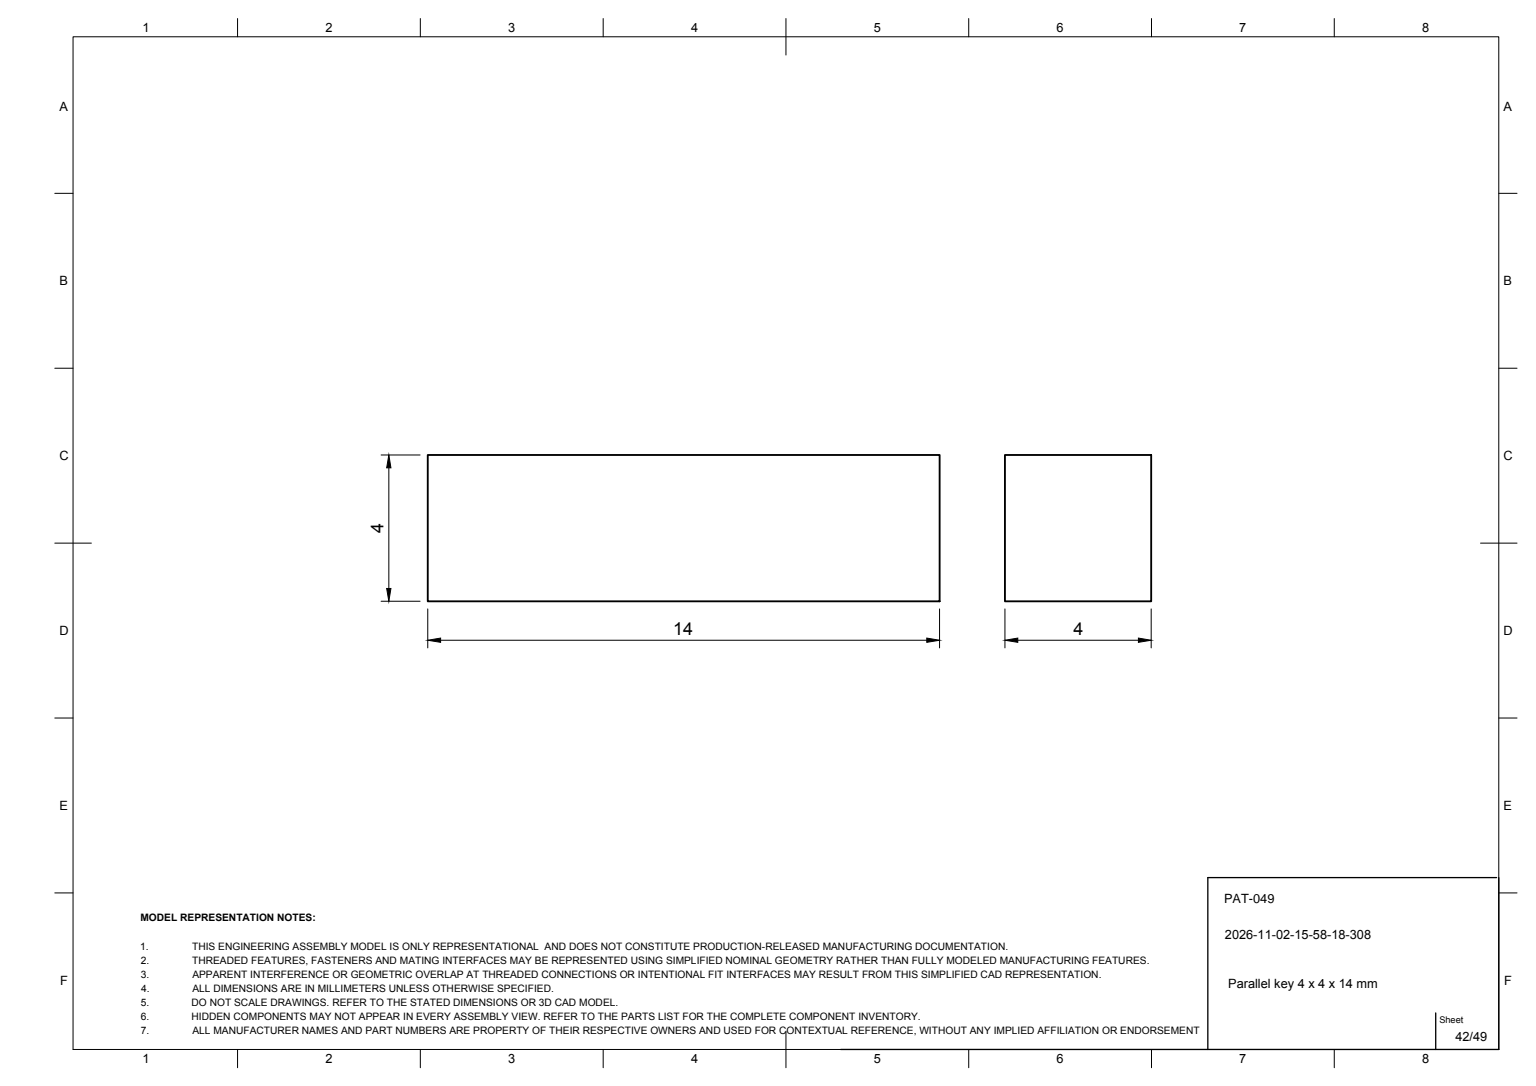
ISO-10303-21;
HEADER;
/* Generated by software containing ST-Developer
 * from STEP Tools, Inc. (www.steptools.com) 
 */

FILE_DESCRIPTION(
/* description */ ('Hand drill press frame (manual)'),
/* implementation_level */ '2;1');

FILE_NAME(
/* name */ 'Parallel key 4 x 4 x 14 mm.step',
/* time_stamp */ '2026-10-28T03:25:28-07:00',
/* author */ (''),
/* organization */ (''),
/* preprocessor_version */ 'ST-DEVELOPER v20.2',
/* originating_system */ 'Autodesk Translation Framework v15.17.0.0',
/* authorisation */ '');

FILE_SCHEMA (('AUTOMOTIVE_DESIGN { 1 0 10303 214 3 1 1 }'));
ENDSEC;

DATA;
#10=MECHANICAL_DESIGN_GEOMETRIC_PRESENTATION_REPRESENTATION('',(#660),#33299);
#563=SHAPE_REPRESENTATION_RELATIONSHIP('SRR','None',#33525,#608);
#608=ADVANCED_BREP_SHAPE_REPRESENTATION('',(#711),#33287);
#660=STYLED_ITEM('',(#33814),#711);
#711=MANIFOLD_SOLID_BREP('Body1',#12679);
#1260=PLANE('',#14070);
#1261=PLANE('',#14071);
#1262=PLANE('',#14072);
#1263=PLANE('',#14073);
#1264=PLANE('',#14074);
#1265=PLANE('',#14075);
#1861=FACE_OUTER_BOUND('',#2697,.T.);
#1862=FACE_OUTER_BOUND('',#2698,.T.);
#1863=FACE_OUTER_BOUND('',#2699,.T.);
#1864=FACE_OUTER_BOUND('',#2700,.T.);
#1865=FACE_OUTER_BOUND('',#2701,.T.);
#1866=FACE_OUTER_BOUND('',#2702,.T.);
#2697=EDGE_LOOP('',(#10979,#10980,#10981,#10982));
#2698=EDGE_LOOP('',(#10983,#10984,#10985,#10986));
#2699=EDGE_LOOP('',(#10987,#10988,#10989,#10990));
#2700=EDGE_LOOP('',(#10991,#10992,#10993,#10994));
#2701=EDGE_LOOP('',(#10995,#10996,#10997,#10998));
#2702=EDGE_LOOP('',(#10999,#11000,#11001,#11002));
#3816=LINE('',#21203,#4981);
#3817=LINE('',#21205,#4982);
#3818=LINE('',#21207,#4983);
#3819=LINE('',#21208,#4984);
#3820=LINE('',#21211,#4985);
#3821=LINE('',#21213,#4986);
#3822=LINE('',#21214,#4987);
#3823=LINE('',#21217,#4988);
#3824=LINE('',#21219,#4989);
#3825=LINE('',#21220,#4990);
#3826=LINE('',#21222,#4991);
#3827=LINE('',#21223,#4992);
#4981=VECTOR('',#17065,1.);
#4982=VECTOR('',#17066,1.);
#4983=VECTOR('',#17067,1.);
#4984=VECTOR('',#17068,1.);
#4985=VECTOR('',#17071,1.);
#4986=VECTOR('',#17072,1.);
#4987=VECTOR('',#17073,1.);
#4988=VECTOR('',#17076,1.);
#4989=VECTOR('',#17077,1.);
#4990=VECTOR('',#17078,1.);
#4991=VECTOR('',#17081,1.);
#4992=VECTOR('',#17082,1.);
#6473=VERTEX_POINT('',#21201);
#6474=VERTEX_POINT('',#21202);
#6475=VERTEX_POINT('',#21204);
#6476=VERTEX_POINT('',#21206);
#6477=VERTEX_POINT('',#21210);
#6478=VERTEX_POINT('',#21212);
#6479=VERTEX_POINT('',#21216);
#6480=VERTEX_POINT('',#21218);
#8018=EDGE_CURVE('',#6473,#6474,#3816,.T.);
#8019=EDGE_CURVE('',#6474,#6475,#3817,.T.);
#8020=EDGE_CURVE('',#6476,#6475,#3818,.T.);
#8021=EDGE_CURVE('',#6473,#6476,#3819,.T.);
#8022=EDGE_CURVE('',#6477,#6473,#3820,.T.);
#8023=EDGE_CURVE('',#6478,#6476,#3821,.T.);
#8024=EDGE_CURVE('',#6477,#6478,#3822,.T.);
#8025=EDGE_CURVE('',#6479,#6477,#3823,.T.);
#8026=EDGE_CURVE('',#6480,#6478,#3824,.T.);
#8027=EDGE_CURVE('',#6479,#6480,#3825,.T.);
#8028=EDGE_CURVE('',#6474,#6479,#3826,.T.);
#8029=EDGE_CURVE('',#6475,#6480,#3827,.T.);
#10979=ORIENTED_EDGE('',*,*,#8018,.T.);
#10980=ORIENTED_EDGE('',*,*,#8019,.T.);
#10981=ORIENTED_EDGE('',*,*,#8020,.F.);
#10982=ORIENTED_EDGE('',*,*,#8021,.F.);
#10983=ORIENTED_EDGE('',*,*,#8022,.T.);
#10984=ORIENTED_EDGE('',*,*,#8021,.T.);
#10985=ORIENTED_EDGE('',*,*,#8023,.F.);
#10986=ORIENTED_EDGE('',*,*,#8024,.F.);
#10987=ORIENTED_EDGE('',*,*,#8025,.T.);
#10988=ORIENTED_EDGE('',*,*,#8024,.T.);
#10989=ORIENTED_EDGE('',*,*,#8026,.F.);
#10990=ORIENTED_EDGE('',*,*,#8027,.F.);
#10991=ORIENTED_EDGE('',*,*,#8028,.T.);
#10992=ORIENTED_EDGE('',*,*,#8027,.T.);
#10993=ORIENTED_EDGE('',*,*,#8029,.F.);
#10994=ORIENTED_EDGE('',*,*,#8019,.F.);
#10995=ORIENTED_EDGE('',*,*,#8029,.T.);
#10996=ORIENTED_EDGE('',*,*,#8026,.T.);
#10997=ORIENTED_EDGE('',*,*,#8023,.T.);
#10998=ORIENTED_EDGE('',*,*,#8020,.T.);
#10999=ORIENTED_EDGE('',*,*,#8028,.F.);
#11000=ORIENTED_EDGE('',*,*,#8018,.F.);
#11001=ORIENTED_EDGE('',*,*,#8022,.F.);
#11002=ORIENTED_EDGE('',*,*,#8025,.F.);
#12470=ADVANCED_FACE('',(#1861),#1260,.T.);
#12471=ADVANCED_FACE('',(#1862),#1261,.T.);
#12472=ADVANCED_FACE('',(#1863),#1262,.T.);
#12473=ADVANCED_FACE('',(#1864),#1263,.T.);
#12474=ADVANCED_FACE('',(#1865),#1264,.T.);
#12475=ADVANCED_FACE('',(#1866),#1265,.F.);
#12679=CLOSED_SHELL('',(#12470,#12471,#12472,#12473,#12474,#12475));
#14069=AXIS2_PLACEMENT_3D('',#21199,#17061,#17062);
#14070=AXIS2_PLACEMENT_3D('',#21200,#17063,#17064);
#14071=AXIS2_PLACEMENT_3D('',#21209,#17069,#17070);
#14072=AXIS2_PLACEMENT_3D('',#21215,#17074,#17075);
#14073=AXIS2_PLACEMENT_3D('',#21221,#17079,#17080);
#14074=AXIS2_PLACEMENT_3D('',#21224,#17083,#17084);
#14075=AXIS2_PLACEMENT_3D('',#21225,#17085,#17086);
#17061=DIRECTION('axis',(0.,0.,1.));
#17062=DIRECTION('refdir',(1.,0.,0.));
#17063=DIRECTION('center_axis',(0.,1.,0.));
#17064=DIRECTION('ref_axis',(-1.,0.,0.));
#17065=DIRECTION('',(-1.,0.,0.));
#17066=DIRECTION('',(0.,0.,1.));
#17067=DIRECTION('',(-1.,0.,0.));
#17068=DIRECTION('',(0.,0.,1.));
#17069=DIRECTION('center_axis',(1.,0.,0.));
#17070=DIRECTION('ref_axis',(0.,1.,0.));
#17071=DIRECTION('',(0.,1.,0.));
#17072=DIRECTION('',(0.,1.,0.));
#17073=DIRECTION('',(0.,0.,1.));
#17074=DIRECTION('center_axis',(0.,-1.,0.));
#17075=DIRECTION('ref_axis',(1.,0.,0.));
#17076=DIRECTION('',(1.,0.,0.));
#17077=DIRECTION('',(1.,0.,0.));
#17078=DIRECTION('',(0.,0.,1.));
#17079=DIRECTION('center_axis',(-1.,0.,0.));
#17080=DIRECTION('ref_axis',(0.,-1.,0.));
#17081=DIRECTION('',(0.,-1.,0.));
#17082=DIRECTION('',(0.,-1.,0.));
#17083=DIRECTION('center_axis',(0.,0.,1.));
#17084=DIRECTION('ref_axis',(1.,0.,0.));
#17085=DIRECTION('center_axis',(0.,0.,1.));
#17086=DIRECTION('ref_axis',(1.,0.,0.));
#21199=CARTESIAN_POINT('',(0.,0.,0.));
#21200=CARTESIAN_POINT('Origin',(-2.5,1.2,19.8));
#21201=CARTESIAN_POINT('',(-2.5,1.2,19.8));
#21202=CARTESIAN_POINT('',(-2.9,1.2,19.8));
#21203=CARTESIAN_POINT('',(-2.5,1.2,19.8));
#21204=CARTESIAN_POINT('',(-2.9,1.2,20.2));
#21205=CARTESIAN_POINT('',(-2.9,1.2,19.8));
#21206=CARTESIAN_POINT('',(-2.5,1.2,20.2));
#21207=CARTESIAN_POINT('',(-2.5,1.2,20.2));
#21208=CARTESIAN_POINT('',(-2.5,1.2,19.8));
#21209=CARTESIAN_POINT('Origin',(-2.5,-0.2,19.8));
#21210=CARTESIAN_POINT('',(-2.5,-0.2,19.8));
#21211=CARTESIAN_POINT('',(-2.5,-0.2,19.8));
#21212=CARTESIAN_POINT('',(-2.5,-0.2,20.2));
#21213=CARTESIAN_POINT('',(-2.5,-0.2,20.2));
#21214=CARTESIAN_POINT('',(-2.5,-0.2,19.8));
#21215=CARTESIAN_POINT('Origin',(-2.9,-0.2,19.8));
#21216=CARTESIAN_POINT('',(-2.9,-0.2,19.8));
#21217=CARTESIAN_POINT('',(-2.9,-0.2,19.8));
#21218=CARTESIAN_POINT('',(-2.9,-0.2,20.2));
#21219=CARTESIAN_POINT('',(-2.9,-0.2,20.2));
#21220=CARTESIAN_POINT('',(-2.9,-0.2,19.8));
#21221=CARTESIAN_POINT('Origin',(-2.9,1.2,19.8));
#21222=CARTESIAN_POINT('',(-2.9,1.2,19.8));
#21223=CARTESIAN_POINT('',(-2.9,1.2,20.2));
#21224=CARTESIAN_POINT('Origin',(-2.7,0.5,20.2));
#21225=CARTESIAN_POINT('Origin',(-2.7,0.5,19.8));
#33235=UNCERTAINTY_MEASURE_WITH_UNIT(LENGTH_MEASURE(0.001),#33300,
'DISTANCE_ACCURACY_VALUE',
'Maximum model space distance between geometric entities at asserted c
onnectivities');
#33247=UNCERTAINTY_MEASURE_WITH_UNIT(LENGTH_MEASURE(0.001),#33300,
'DISTANCE_ACCURACY_VALUE',
'Maximum model space distance between geometric entities at asserted c
onnectivities');
#33287=(
GEOMETRIC_REPRESENTATION_CONTEXT(3)
GLOBAL_UNCERTAINTY_ASSIGNED_CONTEXT((#33235))
GLOBAL_UNIT_ASSIGNED_CONTEXT((#33300,#33302,#33303))
REPRESENTATION_CONTEXT('','3D')
);
#33299=(
GEOMETRIC_REPRESENTATION_CONTEXT(3)
GLOBAL_UNCERTAINTY_ASSIGNED_CONTEXT((#33247))
GLOBAL_UNIT_ASSIGNED_CONTEXT((#33300,#33302,#33303))
REPRESENTATION_CONTEXT('','3D')
);
#33300=(
LENGTH_UNIT()
NAMED_UNIT(*)
SI_UNIT(.CENTI.,.METRE.)
);
#33302=(
NAMED_UNIT(*)
PLANE_ANGLE_UNIT()
SI_UNIT($,.RADIAN.)
);
#33303=(
NAMED_UNIT(*)
SI_UNIT($,.STERADIAN.)
SOLID_ANGLE_UNIT()
);
#33343=SHAPE_DEFINITION_REPRESENTATION(#33405,#33525);
#33405=PRODUCT_DEFINITION_SHAPE('',$,#33577);
#33525=SHAPE_REPRESENTATION('',(#14069),#33287);
#33537=PRODUCT_DEFINITION_CONTEXT('part definition',#33692,'design');
#33577=PRODUCT_DEFINITION('Parallel key 4 x 4 x 14 mm',
'Parallel key 4 x 4 x 14 mm',#33628,#33537);
#33628=PRODUCT_DEFINITION_FORMATION('',$,#33733);
#33692=APPLICATION_CONTEXT(
'Core Data for Automotive Mechanical Design Process');
#33693=PRODUCT_CONTEXT('part definition',#33692,'mechanical');
#33733=PRODUCT('Parallel key 4 x 4 x 14 mm',
'Parallel key 4 x 4 x 14 mm','Parallel key 4 x 4 x 14 mm',(#33693));
#33808=COLOUR_RGB('Grey',0.48,0.52,0.57);
#33809=FILL_AREA_STYLE_COLOUR('',#33808);
#33810=FILL_AREA_STYLE('',(#33809));
#33811=SURFACE_STYLE_FILL_AREA(#33810);
#33812=SURFACE_SIDE_STYLE('',(#33811));
#33813=SURFACE_STYLE_USAGE(.BOTH.,#33812);
#33814=PRESENTATION_STYLE_ASSIGNMENT((#33813));
ENDSEC;
END-ISO-10303-21;
